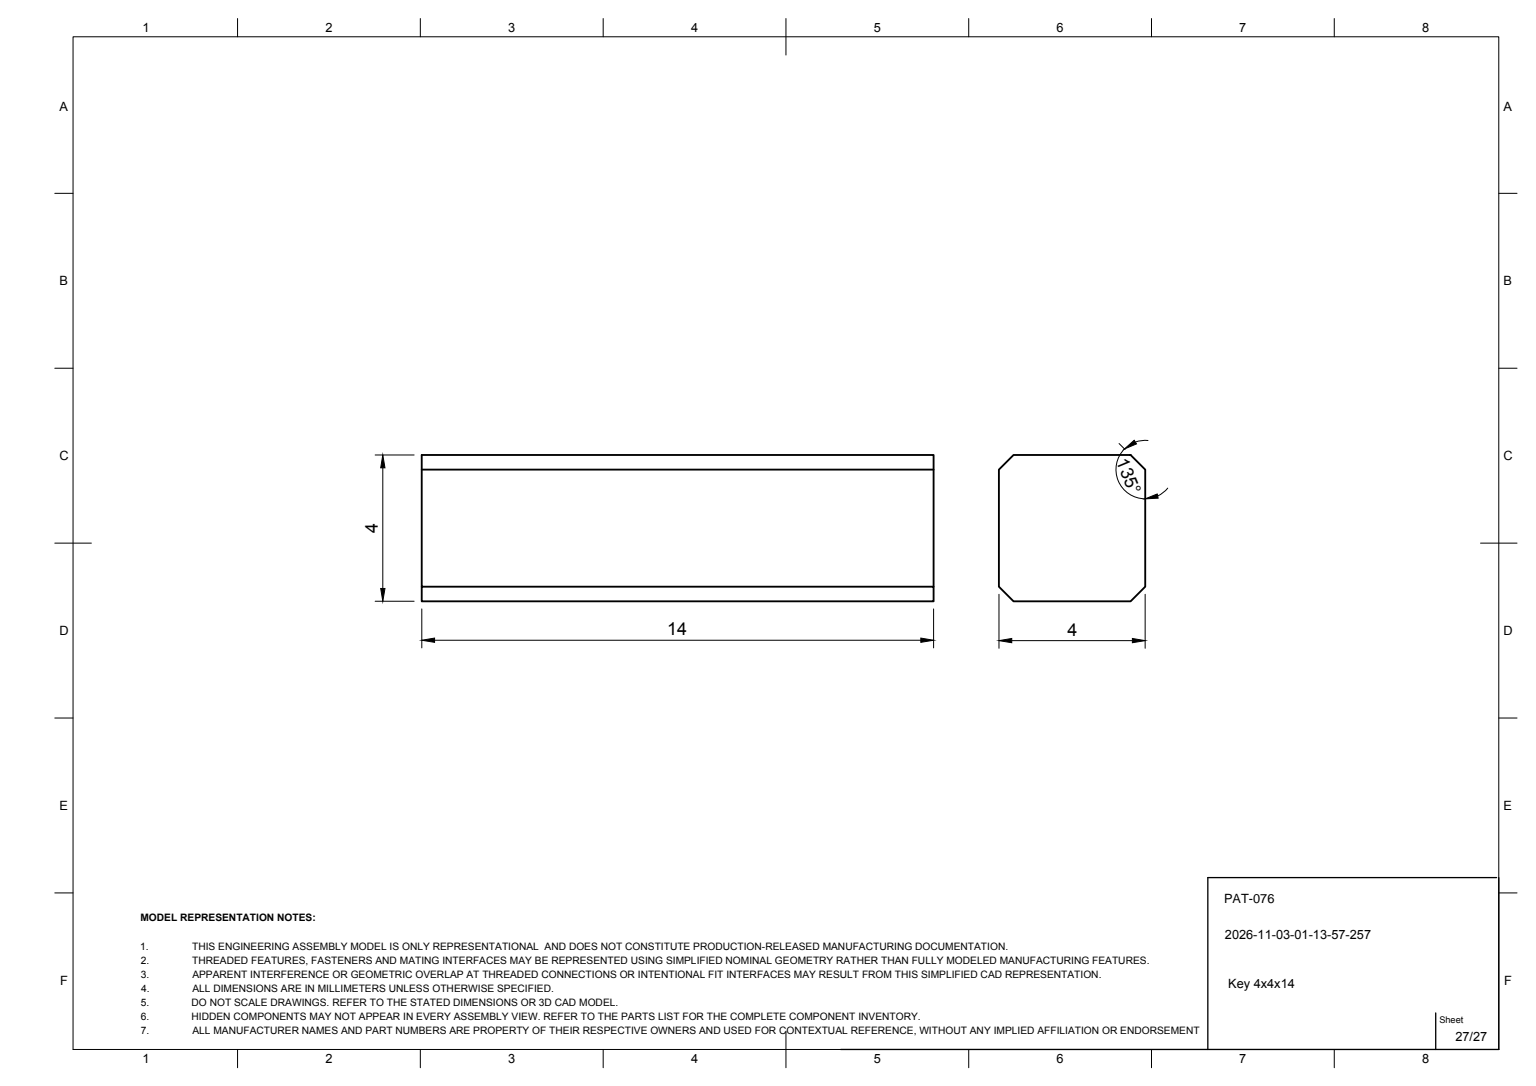
ISO-10303-21;
HEADER;
/* Generated by software containing ST-Developer
 * from STEP Tools, Inc. (www.steptools.com) 
 */

FILE_DESCRIPTION(
/* description */ ('Overhung pulley bearing cartridge'),
/* implementation_level */ '2;1');

FILE_NAME(
/* name */ 'Key 4x4x14.step',
/* time_stamp */ '2026-10-28T03:22:33-07:00',
/* author */ (''),
/* organization */ (''),
/* preprocessor_version */ 'ST-DEVELOPER v20.2',
/* originating_system */ 'Autodesk Translation Framework v15.17.0.0',
/* authorisation */ '');

FILE_SCHEMA (('AUTOMOTIVE_DESIGN { 1 0 10303 214 3 1 1 }'));
ENDSEC;

DATA;
#10=MECHANICAL_DESIGN_GEOMETRIC_PRESENTATION_REPRESENTATION('',(#311),#10963);
#259=SHAPE_REPRESENTATION_RELATIONSHIP('SRR','None',#11081,#281);
#281=ADVANCED_BREP_SHAPE_REPRESENTATION('',(#339),#10961);
#311=STYLED_ITEM('',(#11253),#339);
#339=MANIFOLD_SOLID_BREP('Body1',#5680);
#558=PLANE('',#6651);
#559=PLANE('',#6652);
#560=PLANE('',#6653);
#561=PLANE('',#6654);
#562=PLANE('',#6655);
#563=PLANE('',#6656);
#564=PLANE('',#6657);
#565=PLANE('',#6658);
#566=PLANE('',#6659);
#567=PLANE('',#6660);
#884=FACE_OUTER_BOUND('',#1305,.T.);
#885=FACE_OUTER_BOUND('',#1306,.T.);
#886=FACE_OUTER_BOUND('',#1307,.T.);
#887=FACE_OUTER_BOUND('',#1308,.T.);
#888=FACE_OUTER_BOUND('',#1309,.T.);
#889=FACE_OUTER_BOUND('',#1310,.T.);
#890=FACE_OUTER_BOUND('',#1311,.T.);
#891=FACE_OUTER_BOUND('',#1312,.T.);
#892=FACE_OUTER_BOUND('',#1313,.T.);
#893=FACE_OUTER_BOUND('',#1314,.T.);
#1305=EDGE_LOOP('',(#5069,#5070,#5071,#5072,#5073,#5074,#5075,#5076));
#1306=EDGE_LOOP('',(#5077,#5078,#5079,#5080));
#1307=EDGE_LOOP('',(#5081,#5082,#5083,#5084));
#1308=EDGE_LOOP('',(#5085,#5086,#5087,#5088));
#1309=EDGE_LOOP('',(#5089,#5090,#5091,#5092));
#1310=EDGE_LOOP('',(#5093,#5094,#5095,#5096,#5097,#5098,#5099,#5100));
#1311=EDGE_LOOP('',(#5101,#5102,#5103,#5104));
#1312=EDGE_LOOP('',(#5105,#5106,#5107,#5108));
#1313=EDGE_LOOP('',(#5109,#5110,#5111,#5112));
#1314=EDGE_LOOP('',(#5113,#5114,#5115,#5116));
#1625=LINE('',#10799,#1967);
#1626=LINE('',#10801,#1968);
#1627=LINE('',#10803,#1969);
#1628=LINE('',#10805,#1970);
#1629=LINE('',#10807,#1971);
#1630=LINE('',#10809,#1972);
#1631=LINE('',#10811,#1973);
#1632=LINE('',#10812,#1974);
#1633=LINE('',#10815,#1975);
#1634=LINE('',#10817,#1976);
#1635=LINE('',#10818,#1977);
#1636=LINE('',#10821,#1978);
#1637=LINE('',#10822,#1979);
#1638=LINE('',#10825,#1980);
#1639=LINE('',#10826,#1981);
#1640=LINE('',#10829,#1982);
#1641=LINE('',#10830,#1983);
#1642=LINE('',#10833,#1984);
#1643=LINE('',#10835,#1985);
#1644=LINE('',#10837,#1986);
#1645=LINE('',#10838,#1987);
#1646=LINE('',#10840,#1988);
#1647=LINE('',#10842,#1989);
#1648=LINE('',#10844,#1990);
#1967=VECTOR('',#8439,1.);
#1968=VECTOR('',#8440,1.);
#1969=VECTOR('',#8441,1.);
#1970=VECTOR('',#8442,1.);
#1971=VECTOR('',#8443,1.);
#1972=VECTOR('',#8444,1.);
#1973=VECTOR('',#8445,1.);
#1974=VECTOR('',#8446,1.);
#1975=VECTOR('',#8449,1.);
#1976=VECTOR('',#8450,1.);
#1977=VECTOR('',#8451,1.);
#1978=VECTOR('',#8454,1.);
#1979=VECTOR('',#8455,1.);
#1980=VECTOR('',#8458,1.);
#1981=VECTOR('',#8459,1.);
#1982=VECTOR('',#8462,1.);
#1983=VECTOR('',#8463,1.);
#1984=VECTOR('',#8466,1.);
#1985=VECTOR('',#8467,1.);
#1986=VECTOR('',#8468,1.);
#1987=VECTOR('',#8469,1.);
#1988=VECTOR('',#8472,1.);
#1989=VECTOR('',#8475,1.);
#1990=VECTOR('',#8478,1.);
#2864=VERTEX_POINT('',#10797);
#2865=VERTEX_POINT('',#10798);
#2866=VERTEX_POINT('',#10800);
#2867=VERTEX_POINT('',#10802);
#2868=VERTEX_POINT('',#10804);
#2869=VERTEX_POINT('',#10806);
#2870=VERTEX_POINT('',#10808);
#2871=VERTEX_POINT('',#10810);
#2872=VERTEX_POINT('',#10814);
#2873=VERTEX_POINT('',#10816);
#2874=VERTEX_POINT('',#10820);
#2875=VERTEX_POINT('',#10824);
#2876=VERTEX_POINT('',#10828);
#2877=VERTEX_POINT('',#10832);
#2878=VERTEX_POINT('',#10834);
#2879=VERTEX_POINT('',#10836);
#3604=EDGE_CURVE('',#2864,#2865,#1625,.T.);
#3605=EDGE_CURVE('',#2866,#2864,#1626,.T.);
#3606=EDGE_CURVE('',#2867,#2866,#1627,.T.);
#3607=EDGE_CURVE('',#2868,#2867,#1628,.T.);
#3608=EDGE_CURVE('',#2869,#2868,#1629,.T.);
#3609=EDGE_CURVE('',#2870,#2869,#1630,.T.);
#3610=EDGE_CURVE('',#2871,#2870,#1631,.T.);
#3611=EDGE_CURVE('',#2865,#2871,#1632,.T.);
#3612=EDGE_CURVE('',#2868,#2872,#1633,.T.);
#3613=EDGE_CURVE('',#2872,#2873,#1634,.T.);
#3614=EDGE_CURVE('',#2873,#2869,#1635,.T.);
#3615=EDGE_CURVE('',#2874,#2867,#1636,.T.);
#3616=EDGE_CURVE('',#2874,#2872,#1637,.T.);
#3617=EDGE_CURVE('',#2866,#2875,#1638,.T.);
#3618=EDGE_CURVE('',#2875,#2874,#1639,.T.);
#3619=EDGE_CURVE('',#2876,#2864,#1640,.T.);
#3620=EDGE_CURVE('',#2876,#2875,#1641,.T.);
#3621=EDGE_CURVE('',#2877,#2876,#1642,.T.);
#3622=EDGE_CURVE('',#2878,#2877,#1643,.T.);
#3623=EDGE_CURVE('',#2879,#2878,#1644,.T.);
#3624=EDGE_CURVE('',#2873,#2879,#1645,.T.);
#3625=EDGE_CURVE('',#2865,#2877,#1646,.T.);
#3626=EDGE_CURVE('',#2878,#2871,#1647,.T.);
#3627=EDGE_CURVE('',#2870,#2879,#1648,.T.);
#5069=ORIENTED_EDGE('',*,*,#3604,.F.);
#5070=ORIENTED_EDGE('',*,*,#3605,.F.);
#5071=ORIENTED_EDGE('',*,*,#3606,.F.);
#5072=ORIENTED_EDGE('',*,*,#3607,.F.);
#5073=ORIENTED_EDGE('',*,*,#3608,.F.);
#5074=ORIENTED_EDGE('',*,*,#3609,.F.);
#5075=ORIENTED_EDGE('',*,*,#3610,.F.);
#5076=ORIENTED_EDGE('',*,*,#3611,.F.);
#5077=ORIENTED_EDGE('',*,*,#3608,.T.);
#5078=ORIENTED_EDGE('',*,*,#3612,.T.);
#5079=ORIENTED_EDGE('',*,*,#3613,.T.);
#5080=ORIENTED_EDGE('',*,*,#3614,.T.);
#5081=ORIENTED_EDGE('',*,*,#3607,.T.);
#5082=ORIENTED_EDGE('',*,*,#3615,.F.);
#5083=ORIENTED_EDGE('',*,*,#3616,.T.);
#5084=ORIENTED_EDGE('',*,*,#3612,.F.);
#5085=ORIENTED_EDGE('',*,*,#3606,.T.);
#5086=ORIENTED_EDGE('',*,*,#3617,.T.);
#5087=ORIENTED_EDGE('',*,*,#3618,.T.);
#5088=ORIENTED_EDGE('',*,*,#3615,.T.);
#5089=ORIENTED_EDGE('',*,*,#3605,.T.);
#5090=ORIENTED_EDGE('',*,*,#3619,.F.);
#5091=ORIENTED_EDGE('',*,*,#3620,.T.);
#5092=ORIENTED_EDGE('',*,*,#3617,.F.);
#5093=ORIENTED_EDGE('',*,*,#3613,.F.);
#5094=ORIENTED_EDGE('',*,*,#3616,.F.);
#5095=ORIENTED_EDGE('',*,*,#3618,.F.);
#5096=ORIENTED_EDGE('',*,*,#3620,.F.);
#5097=ORIENTED_EDGE('',*,*,#3621,.F.);
#5098=ORIENTED_EDGE('',*,*,#3622,.F.);
#5099=ORIENTED_EDGE('',*,*,#3623,.F.);
#5100=ORIENTED_EDGE('',*,*,#3624,.F.);
#5101=ORIENTED_EDGE('',*,*,#3604,.T.);
#5102=ORIENTED_EDGE('',*,*,#3625,.T.);
#5103=ORIENTED_EDGE('',*,*,#3621,.T.);
#5104=ORIENTED_EDGE('',*,*,#3619,.T.);
#5105=ORIENTED_EDGE('',*,*,#3611,.T.);
#5106=ORIENTED_EDGE('',*,*,#3626,.F.);
#5107=ORIENTED_EDGE('',*,*,#3622,.T.);
#5108=ORIENTED_EDGE('',*,*,#3625,.F.);
#5109=ORIENTED_EDGE('',*,*,#3610,.T.);
#5110=ORIENTED_EDGE('',*,*,#3627,.T.);
#5111=ORIENTED_EDGE('',*,*,#3623,.T.);
#5112=ORIENTED_EDGE('',*,*,#3626,.T.);
#5113=ORIENTED_EDGE('',*,*,#3609,.T.);
#5114=ORIENTED_EDGE('',*,*,#3614,.F.);
#5115=ORIENTED_EDGE('',*,*,#3624,.T.);
#5116=ORIENTED_EDGE('',*,*,#3627,.F.);
#5628=ADVANCED_FACE('',(#884),#558,.T.);
#5629=ADVANCED_FACE('',(#885),#559,.T.);
#5630=ADVANCED_FACE('',(#886),#560,.T.);
#5631=ADVANCED_FACE('',(#887),#561,.T.);
#5632=ADVANCED_FACE('',(#888),#562,.T.);
#5633=ADVANCED_FACE('',(#889),#563,.F.);
#5634=ADVANCED_FACE('',(#890),#564,.T.);
#5635=ADVANCED_FACE('',(#891),#565,.T.);
#5636=ADVANCED_FACE('',(#892),#566,.T.);
#5637=ADVANCED_FACE('',(#893),#567,.F.);
#5680=CLOSED_SHELL('',(#5628,#5629,#5630,#5631,#5632,#5633,#5634,#5635,
#5636,#5637));
#6650=AXIS2_PLACEMENT_3D('',#10795,#8435,#8436);
#6651=AXIS2_PLACEMENT_3D('',#10796,#8437,#8438);
#6652=AXIS2_PLACEMENT_3D('',#10813,#8447,#8448);
#6653=AXIS2_PLACEMENT_3D('',#10819,#8452,#8453);
#6654=AXIS2_PLACEMENT_3D('',#10823,#8456,#8457);
#6655=AXIS2_PLACEMENT_3D('',#10827,#8460,#8461);
#6656=AXIS2_PLACEMENT_3D('',#10831,#8464,#8465);
#6657=AXIS2_PLACEMENT_3D('',#10839,#8470,#8471);
#6658=AXIS2_PLACEMENT_3D('',#10841,#8473,#8474);
#6659=AXIS2_PLACEMENT_3D('',#10843,#8476,#8477);
#6660=AXIS2_PLACEMENT_3D('',#10845,#8479,#8480);
#8435=DIRECTION('axis',(0.,0.,1.));
#8436=DIRECTION('refdir',(1.,0.,0.));
#8437=DIRECTION('center_axis',(1.,0.,0.));
#8438=DIRECTION('ref_axis',(0.,0.,-1.));
#8439=DIRECTION('',(0.,0.707106781186547,-0.707106781186548));
#8440=DIRECTION('',(0.,1.,0.));
#8441=DIRECTION('',(0.,0.707106781186547,0.707106781186548));
#8442=DIRECTION('',(0.,0.,1.));
#8443=DIRECTION('',(0.,-0.707106781186548,0.707106781186548));
#8444=DIRECTION('',(0.,-1.,0.));
#8445=DIRECTION('',(0.,-0.707106781186548,-0.707106781186548));
#8446=DIRECTION('',(0.,0.,-1.));
#8447=DIRECTION('center_axis',(0.,-0.707106781186548,-0.707106781186548));
#8448=DIRECTION('ref_axis',(-1.,0.,0.));
#8449=DIRECTION('',(-1.,0.,0.));
#8450=DIRECTION('',(0.,0.707106781186548,-0.707106781186548));
#8451=DIRECTION('',(1.,0.,0.));
#8452=DIRECTION('center_axis',(0.,-1.,0.));
#8453=DIRECTION('ref_axis',(1.,0.,0.));
#8454=DIRECTION('',(1.,0.,0.));
#8455=DIRECTION('',(0.,0.,-1.));
#8456=DIRECTION('center_axis',(0.,-0.707106781186548,0.707106781186547));
#8457=DIRECTION('ref_axis',(1.,0.,0.));
#8458=DIRECTION('',(-1.,0.,0.));
#8459=DIRECTION('',(0.,-0.707106781186547,-0.707106781186548));
#8460=DIRECTION('center_axis',(0.,0.,1.));
#8461=DIRECTION('ref_axis',(1.,0.,0.));
#8462=DIRECTION('',(1.,0.,0.));
#8463=DIRECTION('',(0.,-1.,0.));
#8464=DIRECTION('center_axis',(1.,0.,0.));
#8465=DIRECTION('ref_axis',(0.,0.,-1.));
#8466=DIRECTION('',(0.,-0.707106781186547,0.707106781186548));
#8467=DIRECTION('',(0.,0.,1.));
#8468=DIRECTION('',(0.,0.707106781186548,0.707106781186548));
#8469=DIRECTION('',(0.,1.,0.));
#8470=DIRECTION('center_axis',(0.,0.707106781186548,0.707106781186547));
#8471=DIRECTION('ref_axis',(1.,0.,0.));
#8472=DIRECTION('',(-1.,0.,0.));
#8473=DIRECTION('center_axis',(0.,1.,0.));
#8474=DIRECTION('ref_axis',(-1.,0.,0.));
#8475=DIRECTION('',(1.,0.,0.));
#8476=DIRECTION('center_axis',(0.,0.707106781186548,-0.707106781186548));
#8477=DIRECTION('ref_axis',(-1.,0.,0.));
#8478=DIRECTION('',(-1.,0.,0.));
#8479=DIRECTION('center_axis',(0.,0.,1.));
#8480=DIRECTION('ref_axis',(1.,0.,0.));
#10795=CARTESIAN_POINT('',(0.,0.,0.));
#10796=CARTESIAN_POINT('Origin',(0.7,0.,0.25));
#10797=CARTESIAN_POINT('',(0.7,0.16,0.4));
#10798=CARTESIAN_POINT('',(0.7,0.2,0.36));
#10799=CARTESIAN_POINT('',(0.7,0.1675,0.3925));
#10800=CARTESIAN_POINT('',(0.7,-0.16,0.4));
#10801=CARTESIAN_POINT('',(0.7,0.,0.4));
#10802=CARTESIAN_POINT('',(0.7,-0.2,0.36));
#10803=CARTESIAN_POINT('',(0.7,-0.1675,0.3925));
#10804=CARTESIAN_POINT('',(0.7,-0.2,0.04));
#10805=CARTESIAN_POINT('',(0.7,-0.2,0.125));
#10806=CARTESIAN_POINT('',(0.7,-0.16,0.));
#10807=CARTESIAN_POINT('',(0.7,-0.1925,0.0325));
#10808=CARTESIAN_POINT('',(0.7,0.16,0.));
#10809=CARTESIAN_POINT('',(0.7,0.,0.));
#10810=CARTESIAN_POINT('',(0.7,0.2,0.04));
#10811=CARTESIAN_POINT('',(0.7,0.1925,0.0325));
#10812=CARTESIAN_POINT('',(0.7,0.2,0.125));
#10813=CARTESIAN_POINT('Origin',(-0.4,-0.18,0.02));
#10814=CARTESIAN_POINT('',(-0.7,-0.2,0.04));
#10815=CARTESIAN_POINT('',(-0.4,-0.2,0.04));
#10816=CARTESIAN_POINT('',(-0.7,-0.16,0.));
#10817=CARTESIAN_POINT('',(-0.7,-0.1925,0.0325));
#10818=CARTESIAN_POINT('',(-0.4,-0.16,0.));
#10819=CARTESIAN_POINT('Origin',(-0.8,-0.2,0.));
#10820=CARTESIAN_POINT('',(-0.7,-0.2,0.36));
#10821=CARTESIAN_POINT('',(-0.4,-0.2,0.36));
#10822=CARTESIAN_POINT('',(-0.7,-0.2,0.125));
#10823=CARTESIAN_POINT('Origin',(-0.4,-0.18,0.38));
#10824=CARTESIAN_POINT('',(-0.7,-0.16,0.4));
#10825=CARTESIAN_POINT('',(-0.4,-0.16,0.4));
#10826=CARTESIAN_POINT('',(-0.7,-0.1675,0.3925));
#10827=CARTESIAN_POINT('Origin',(0.,0.,0.4));
#10828=CARTESIAN_POINT('',(-0.7,0.16,0.4));
#10829=CARTESIAN_POINT('',(0.4,0.16,0.4));
#10830=CARTESIAN_POINT('',(-0.7,0.,0.4));
#10831=CARTESIAN_POINT('Origin',(-0.7,0.,0.25));
#10832=CARTESIAN_POINT('',(-0.7,0.2,0.36));
#10833=CARTESIAN_POINT('',(-0.7,0.1675,0.3925));
#10834=CARTESIAN_POINT('',(-0.7,0.2,0.04));
#10835=CARTESIAN_POINT('',(-0.7,0.2,0.125));
#10836=CARTESIAN_POINT('',(-0.7,0.16,0.));
#10837=CARTESIAN_POINT('',(-0.7,0.1925,0.0325));
#10838=CARTESIAN_POINT('',(-0.7,0.,0.));
#10839=CARTESIAN_POINT('Origin',(0.4,0.18,0.38));
#10840=CARTESIAN_POINT('',(0.4,0.2,0.36));
#10841=CARTESIAN_POINT('Origin',(0.8,0.2,0.));
#10842=CARTESIAN_POINT('',(0.4,0.2,0.04));
#10843=CARTESIAN_POINT('Origin',(0.4,0.18,0.02));
#10844=CARTESIAN_POINT('',(0.4,0.16,0.));
#10845=CARTESIAN_POINT('Origin',(0.,0.,0.));
#10934=UNCERTAINTY_MEASURE_WITH_UNIT(LENGTH_MEASURE(0.001),#10964,
'DISTANCE_ACCURACY_VALUE',
'Maximum model space distance between geometric entities at asserted c
onnectivities');
#10936=UNCERTAINTY_MEASURE_WITH_UNIT(LENGTH_MEASURE(0.001),#10964,
'DISTANCE_ACCURACY_VALUE',
'Maximum model space distance between geometric entities at asserted c
onnectivities');
#10961=(
GEOMETRIC_REPRESENTATION_CONTEXT(3)
GLOBAL_UNCERTAINTY_ASSIGNED_CONTEXT((#10934))
GLOBAL_UNIT_ASSIGNED_CONTEXT((#10964,#10966,#10967))
REPRESENTATION_CONTEXT('','3D')
);
#10963=(
GEOMETRIC_REPRESENTATION_CONTEXT(3)
GLOBAL_UNCERTAINTY_ASSIGNED_CONTEXT((#10936))
GLOBAL_UNIT_ASSIGNED_CONTEXT((#10964,#10966,#10967))
REPRESENTATION_CONTEXT('','3D')
);
#10964=(
LENGTH_UNIT()
NAMED_UNIT(*)
SI_UNIT(.CENTI.,.METRE.)
);
#10966=(
NAMED_UNIT(*)
PLANE_ANGLE_UNIT()
SI_UNIT($,.RADIAN.)
);
#10967=(
NAMED_UNIT(*)
SI_UNIT($,.STERADIAN.)
SOLID_ANGLE_UNIT()
);
#10992=SHAPE_DEFINITION_REPRESENTATION(#11045,#11081);
#11045=PRODUCT_DEFINITION_SHAPE('',$,#11108);
#11081=SHAPE_REPRESENTATION('',(#6650),#10961);
#11083=PRODUCT_DEFINITION_CONTEXT('part definition',#11163,'design');
#11108=PRODUCT_DEFINITION('Key 4x4x14','Key 4x4x14',#11134,#11083);
#11134=PRODUCT_DEFINITION_FORMATION('',$,#11189);
#11163=APPLICATION_CONTEXT(
'Core Data for Automotive Mechanical Design Process');
#11164=PRODUCT_CONTEXT('part definition',#11163,'mechanical');
#11189=PRODUCT('Key 4x4x14','Key 4x4x14','Key 4x4x14',(#11164));
#11247=COLOUR_RGB('Grey',0.48,0.52,0.57);
#11248=FILL_AREA_STYLE_COLOUR('',#11247);
#11249=FILL_AREA_STYLE('',(#11248));
#11250=SURFACE_STYLE_FILL_AREA(#11249);
#11251=SURFACE_SIDE_STYLE('',(#11250));
#11252=SURFACE_STYLE_USAGE(.BOTH.,#11251);
#11253=PRESENTATION_STYLE_ASSIGNMENT((#11252));
ENDSEC;
END-ISO-10303-21;
